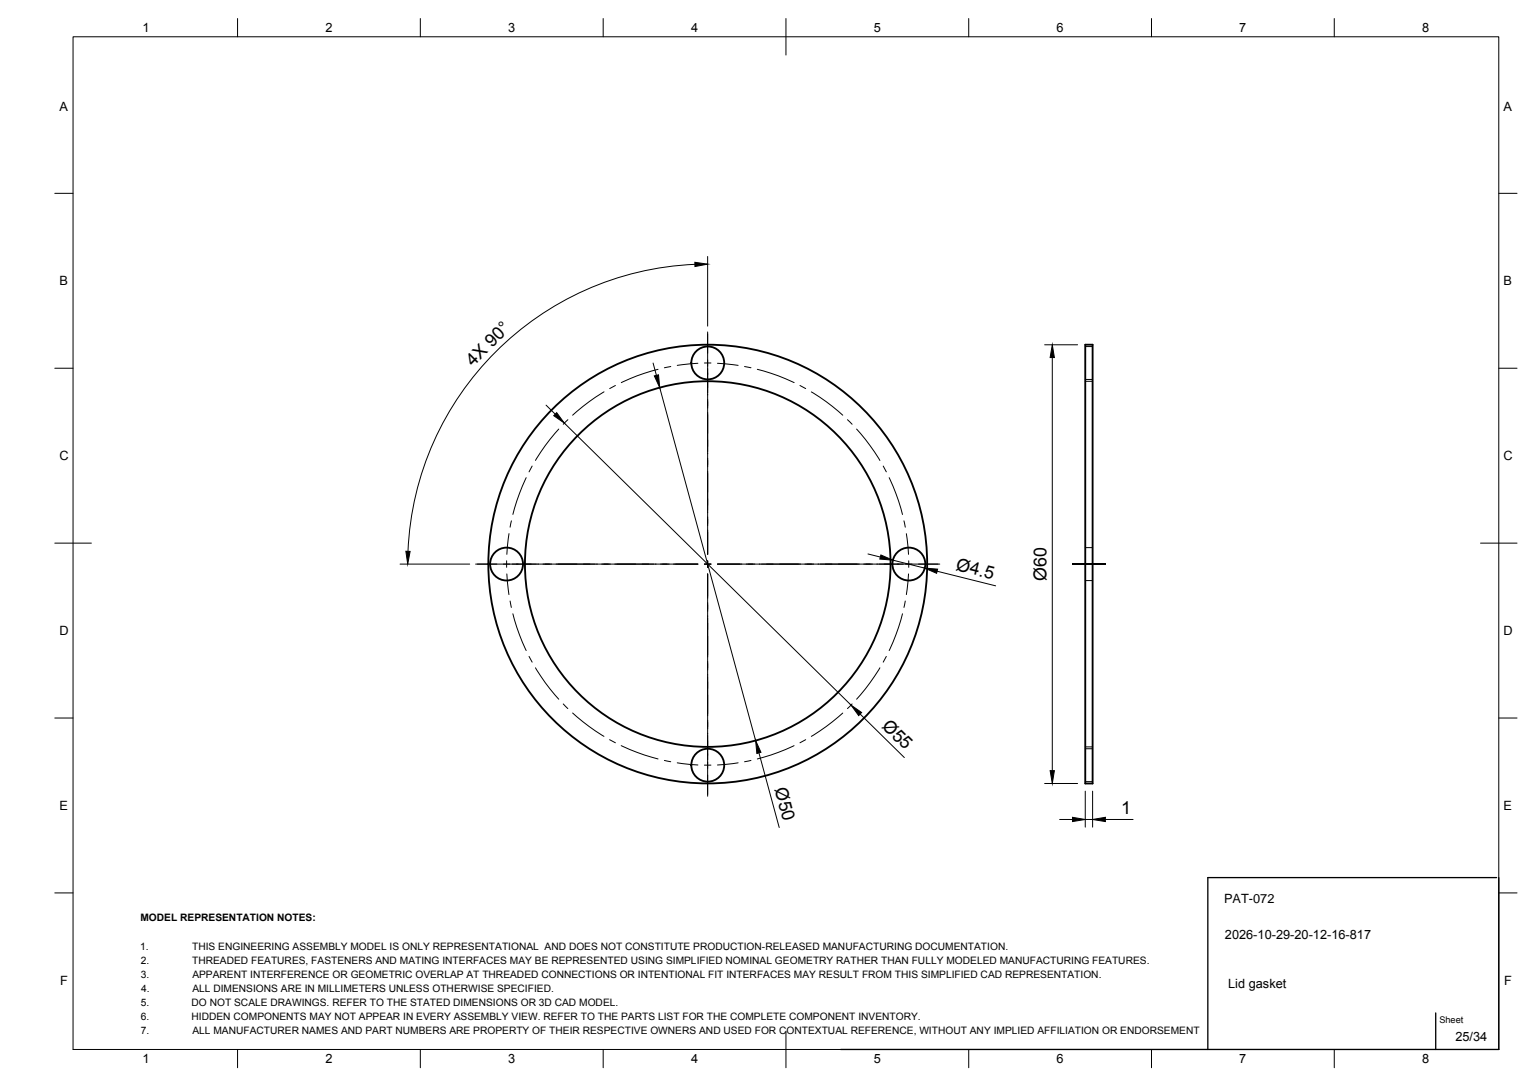
ISO-10303-21;
HEADER;
/* Generated by software containing ST-Developer
 * from STEP Tools, Inc. (www.steptools.com) 
 */

FILE_DESCRIPTION(
/* description */ ('PAT-072'),
/* implementation_level */ '2;1');

FILE_NAME(
/* name */ 'Lid gasket.step',
/* time_stamp */ '2026-10-29T20:11:56-07:00',
/* author */ (''),
/* organization */ (''),
/* preprocessor_version */ 'ST-DEVELOPER v20.2',
/* originating_system */ 'Autodesk Translation Framework v15.17.0.0',
/* authorisation */ '');

FILE_SCHEMA (('AUTOMOTIVE_DESIGN { 1 0 10303 214 3 1 1 }'));
ENDSEC;

DATA;
#10=MECHANICAL_DESIGN_GEOMETRIC_PRESENTATION_REPRESENTATION('',(#358),#11432);
#286=SHAPE_REPRESENTATION_RELATIONSHIP('SRR','None',#11590,#322);
#322=ADVANCED_BREP_SHAPE_REPRESENTATION('',(#394),#11421);
#358=STYLED_ITEM('',(#11833),#394);
#394=MANIFOLD_SOLID_BREP('Body1',#6093);
#532=FACE_BOUND('',#1572,.T.);
#533=FACE_BOUND('',#1573,.T.);
#534=FACE_BOUND('',#1574,.T.);
#535=FACE_BOUND('',#1575,.T.);
#536=FACE_BOUND('',#1576,.T.);
#537=FACE_BOUND('',#1578,.T.);
#538=FACE_BOUND('',#1579,.T.);
#539=FACE_BOUND('',#1580,.T.);
#540=FACE_BOUND('',#1581,.T.);
#541=FACE_BOUND('',#1582,.T.);
#730=PLANE('',#7043);
#731=PLANE('',#7044);
#1063=FACE_OUTER_BOUND('',#1565,.T.);
#1064=FACE_OUTER_BOUND('',#1566,.T.);
#1065=FACE_OUTER_BOUND('',#1567,.T.);
#1066=FACE_OUTER_BOUND('',#1568,.T.);
#1067=FACE_OUTER_BOUND('',#1569,.T.);
#1068=FACE_OUTER_BOUND('',#1570,.T.);
#1069=FACE_OUTER_BOUND('',#1571,.T.);
#1070=FACE_OUTER_BOUND('',#1577,.T.);
#1565=EDGE_LOOP('',(#5150,#5151,#5152,#5153));
#1566=EDGE_LOOP('',(#5154,#5155,#5156,#5157));
#1567=EDGE_LOOP('',(#5158,#5159,#5160,#5161));
#1568=EDGE_LOOP('',(#5162,#5163,#5164,#5165));
#1569=EDGE_LOOP('',(#5166,#5167,#5168,#5169));
#1570=EDGE_LOOP('',(#5170,#5171,#5172,#5173));
#1571=EDGE_LOOP('',(#5174));
#1572=EDGE_LOOP('',(#5175));
#1573=EDGE_LOOP('',(#5176));
#1574=EDGE_LOOP('',(#5177));
#1575=EDGE_LOOP('',(#5178));
#1576=EDGE_LOOP('',(#5179));
#1577=EDGE_LOOP('',(#5180));
#1578=EDGE_LOOP('',(#5181));
#1579=EDGE_LOOP('',(#5182));
#1580=EDGE_LOOP('',(#5183));
#1581=EDGE_LOOP('',(#5184));
#1582=EDGE_LOOP('',(#5185));
#1992=LINE('',#10857,#2411);
#1993=LINE('',#10863,#2412);
#1994=LINE('',#10869,#2413);
#1995=LINE('',#10875,#2414);
#1996=LINE('',#10881,#2415);
#1997=LINE('',#10887,#2416);
#2411=VECTOR('',#8593,0.225);
#2412=VECTOR('',#8600,0.225);
#2413=VECTOR('',#8607,0.225);
#2414=VECTOR('',#8614,0.225);
#2415=VECTOR('',#8621,2.5);
#2416=VECTOR('',#8628,3.);
#2767=CIRCLE('',#7026,0.225);
#2768=CIRCLE('',#7027,0.225);
#2769=CIRCLE('',#7029,0.225);
#2770=CIRCLE('',#7030,0.225);
#2771=CIRCLE('',#7032,0.225);
#2772=CIRCLE('',#7033,0.225);
#2773=CIRCLE('',#7035,0.225);
#2774=CIRCLE('',#7036,0.225);
#2775=CIRCLE('',#7038,2.5);
#2776=CIRCLE('',#7039,2.5);
#2777=CIRCLE('',#7041,3.);
#2778=CIRCLE('',#7042,3.);
#3190=VERTEX_POINT('',#10854);
#3191=VERTEX_POINT('',#10856);
#3192=VERTEX_POINT('',#10860);
#3193=VERTEX_POINT('',#10862);
#3194=VERTEX_POINT('',#10866);
#3195=VERTEX_POINT('',#10868);
#3196=VERTEX_POINT('',#10872);
#3197=VERTEX_POINT('',#10874);
#3198=VERTEX_POINT('',#10878);
#3199=VERTEX_POINT('',#10880);
#3200=VERTEX_POINT('',#10884);
#3201=VERTEX_POINT('',#10886);
#3864=EDGE_CURVE('',#3190,#3190,#2767,.T.);
#3865=EDGE_CURVE('',#3190,#3191,#1992,.T.);
#3866=EDGE_CURVE('',#3191,#3191,#2768,.T.);
#3867=EDGE_CURVE('',#3192,#3192,#2769,.T.);
#3868=EDGE_CURVE('',#3192,#3193,#1993,.T.);
#3869=EDGE_CURVE('',#3193,#3193,#2770,.T.);
#3870=EDGE_CURVE('',#3194,#3194,#2771,.T.);
#3871=EDGE_CURVE('',#3194,#3195,#1994,.T.);
#3872=EDGE_CURVE('',#3195,#3195,#2772,.T.);
#3873=EDGE_CURVE('',#3196,#3196,#2773,.T.);
#3874=EDGE_CURVE('',#3196,#3197,#1995,.T.);
#3875=EDGE_CURVE('',#3197,#3197,#2774,.T.);
#3876=EDGE_CURVE('',#3198,#3198,#2775,.T.);
#3877=EDGE_CURVE('',#3198,#3199,#1996,.T.);
#3878=EDGE_CURVE('',#3199,#3199,#2776,.T.);
#3879=EDGE_CURVE('',#3200,#3200,#2777,.T.);
#3880=EDGE_CURVE('',#3200,#3201,#1997,.T.);
#3881=EDGE_CURVE('',#3201,#3201,#2778,.T.);
#5150=ORIENTED_EDGE('',*,*,#3864,.F.);
#5151=ORIENTED_EDGE('',*,*,#3865,.T.);
#5152=ORIENTED_EDGE('',*,*,#3866,.F.);
#5153=ORIENTED_EDGE('',*,*,#3865,.F.);
#5154=ORIENTED_EDGE('',*,*,#3867,.F.);
#5155=ORIENTED_EDGE('',*,*,#3868,.T.);
#5156=ORIENTED_EDGE('',*,*,#3869,.F.);
#5157=ORIENTED_EDGE('',*,*,#3868,.F.);
#5158=ORIENTED_EDGE('',*,*,#3870,.F.);
#5159=ORIENTED_EDGE('',*,*,#3871,.T.);
#5160=ORIENTED_EDGE('',*,*,#3872,.F.);
#5161=ORIENTED_EDGE('',*,*,#3871,.F.);
#5162=ORIENTED_EDGE('',*,*,#3873,.F.);
#5163=ORIENTED_EDGE('',*,*,#3874,.T.);
#5164=ORIENTED_EDGE('',*,*,#3875,.F.);
#5165=ORIENTED_EDGE('',*,*,#3874,.F.);
#5166=ORIENTED_EDGE('',*,*,#3876,.F.);
#5167=ORIENTED_EDGE('',*,*,#3877,.T.);
#5168=ORIENTED_EDGE('',*,*,#3878,.T.);
#5169=ORIENTED_EDGE('',*,*,#3877,.F.);
#5170=ORIENTED_EDGE('',*,*,#3879,.F.);
#5171=ORIENTED_EDGE('',*,*,#3880,.T.);
#5172=ORIENTED_EDGE('',*,*,#3881,.T.);
#5173=ORIENTED_EDGE('',*,*,#3880,.F.);
#5174=ORIENTED_EDGE('',*,*,#3879,.T.);
#5175=ORIENTED_EDGE('',*,*,#3876,.T.);
#5176=ORIENTED_EDGE('',*,*,#3875,.T.);
#5177=ORIENTED_EDGE('',*,*,#3872,.T.);
#5178=ORIENTED_EDGE('',*,*,#3869,.T.);
#5179=ORIENTED_EDGE('',*,*,#3866,.T.);
#5180=ORIENTED_EDGE('',*,*,#3881,.F.);
#5181=ORIENTED_EDGE('',*,*,#3878,.F.);
#5182=ORIENTED_EDGE('',*,*,#3873,.T.);
#5183=ORIENTED_EDGE('',*,*,#3870,.T.);
#5184=ORIENTED_EDGE('',*,*,#3867,.T.);
#5185=ORIENTED_EDGE('',*,*,#3864,.T.);
#5665=CYLINDRICAL_SURFACE('',#7025,0.225);
#5666=CYLINDRICAL_SURFACE('',#7028,0.225);
#5667=CYLINDRICAL_SURFACE('',#7031,0.225);
#5668=CYLINDRICAL_SURFACE('',#7034,0.225);
#5669=CYLINDRICAL_SURFACE('',#7037,2.5);
#5670=CYLINDRICAL_SURFACE('',#7040,3.);
#5962=ADVANCED_FACE('',(#1063),#5665,.F.);
#5963=ADVANCED_FACE('',(#1064),#5666,.F.);
#5964=ADVANCED_FACE('',(#1065),#5667,.F.);
#5965=ADVANCED_FACE('',(#1066),#5668,.F.);
#5966=ADVANCED_FACE('',(#1067),#5669,.F.);
#5967=ADVANCED_FACE('',(#1068),#5670,.T.);
#5968=ADVANCED_FACE('',(#1069,#532,#533,#534,#535,#536),#730,.T.);
#5969=ADVANCED_FACE('',(#1070,#537,#538,#539,#540,#541),#731,.F.);
#6093=CLOSED_SHELL('',(#5962,#5963,#5964,#5965,#5966,#5967,#5968,#5969));
#7024=AXIS2_PLACEMENT_3D('',#10852,#8587,#8588);
#7025=AXIS2_PLACEMENT_3D('',#10853,#8589,#8590);
#7026=AXIS2_PLACEMENT_3D('',#10855,#8591,#8592);
#7027=AXIS2_PLACEMENT_3D('',#10858,#8594,#8595);
#7028=AXIS2_PLACEMENT_3D('',#10859,#8596,#8597);
#7029=AXIS2_PLACEMENT_3D('',#10861,#8598,#8599);
#7030=AXIS2_PLACEMENT_3D('',#10864,#8601,#8602);
#7031=AXIS2_PLACEMENT_3D('',#10865,#8603,#8604);
#7032=AXIS2_PLACEMENT_3D('',#10867,#8605,#8606);
#7033=AXIS2_PLACEMENT_3D('',#10870,#8608,#8609);
#7034=AXIS2_PLACEMENT_3D('',#10871,#8610,#8611);
#7035=AXIS2_PLACEMENT_3D('',#10873,#8612,#8613);
#7036=AXIS2_PLACEMENT_3D('',#10876,#8615,#8616);
#7037=AXIS2_PLACEMENT_3D('',#10877,#8617,#8618);
#7038=AXIS2_PLACEMENT_3D('',#10879,#8619,#8620);
#7039=AXIS2_PLACEMENT_3D('',#10882,#8622,#8623);
#7040=AXIS2_PLACEMENT_3D('',#10883,#8624,#8625);
#7041=AXIS2_PLACEMENT_3D('',#10885,#8626,#8627);
#7042=AXIS2_PLACEMENT_3D('',#10888,#8629,#8630);
#7043=AXIS2_PLACEMENT_3D('',#10889,#8631,#8632);
#7044=AXIS2_PLACEMENT_3D('',#10890,#8633,#8634);
#8587=DIRECTION('axis',(0.,0.,1.));
#8588=DIRECTION('refdir',(1.,0.,0.));
#8589=DIRECTION('center_axis',(0.,0.,1.));
#8590=DIRECTION('ref_axis',(1.,0.,0.));
#8591=DIRECTION('center_axis',(0.,0.,1.));
#8592=DIRECTION('ref_axis',(1.,0.,0.));
#8593=DIRECTION('',(0.,0.,1.));
#8594=DIRECTION('center_axis',(0.,0.,-1.));
#8595=DIRECTION('ref_axis',(1.,0.,0.));
#8596=DIRECTION('center_axis',(0.,0.,1.));
#8597=DIRECTION('ref_axis',(1.,0.,0.));
#8598=DIRECTION('center_axis',(0.,0.,1.));
#8599=DIRECTION('ref_axis',(1.,0.,0.));
#8600=DIRECTION('',(0.,0.,1.));
#8601=DIRECTION('center_axis',(0.,0.,-1.));
#8602=DIRECTION('ref_axis',(1.,0.,0.));
#8603=DIRECTION('center_axis',(0.,0.,1.));
#8604=DIRECTION('ref_axis',(1.,0.,0.));
#8605=DIRECTION('center_axis',(0.,0.,1.));
#8606=DIRECTION('ref_axis',(1.,0.,0.));
#8607=DIRECTION('',(0.,0.,1.));
#8608=DIRECTION('center_axis',(0.,0.,-1.));
#8609=DIRECTION('ref_axis',(1.,0.,0.));
#8610=DIRECTION('center_axis',(0.,0.,1.));
#8611=DIRECTION('ref_axis',(1.,0.,0.));
#8612=DIRECTION('center_axis',(0.,0.,1.));
#8613=DIRECTION('ref_axis',(1.,0.,0.));
#8614=DIRECTION('',(0.,0.,1.));
#8615=DIRECTION('center_axis',(0.,0.,-1.));
#8616=DIRECTION('ref_axis',(1.,0.,0.));
#8617=DIRECTION('center_axis',(0.,0.,1.));
#8618=DIRECTION('ref_axis',(1.,0.,0.));
#8619=DIRECTION('center_axis',(0.,0.,-1.));
#8620=DIRECTION('ref_axis',(1.,0.,0.));
#8621=DIRECTION('',(0.,0.,-1.));
#8622=DIRECTION('center_axis',(0.,0.,-1.));
#8623=DIRECTION('ref_axis',(1.,0.,0.));
#8624=DIRECTION('center_axis',(0.,0.,1.));
#8625=DIRECTION('ref_axis',(1.,0.,0.));
#8626=DIRECTION('center_axis',(0.,0.,1.));
#8627=DIRECTION('ref_axis',(1.,0.,0.));
#8628=DIRECTION('',(0.,0.,-1.));
#8629=DIRECTION('center_axis',(0.,0.,1.));
#8630=DIRECTION('ref_axis',(1.,0.,0.));
#8631=DIRECTION('center_axis',(0.,0.,1.));
#8632=DIRECTION('ref_axis',(1.,0.,0.));
#8633=DIRECTION('center_axis',(0.,0.,1.));
#8634=DIRECTION('ref_axis',(1.,0.,0.));
#10852=CARTESIAN_POINT('',(0.,0.,0.));
#10853=CARTESIAN_POINT('Origin',(-2.75,3.36777869765522E-16,14.9));
#10854=CARTESIAN_POINT('',(-2.975,3.09223316784707E-16,15.));
#10855=CARTESIAN_POINT('Origin',(-2.75,3.36777869765522E-16,15.));
#10856=CARTESIAN_POINT('',(-2.975,3.64332422746338E-16,15.1));
#10857=CARTESIAN_POINT('',(-2.975,3.09223316784707E-16,14.9));
#10858=CARTESIAN_POINT('Origin',(-2.75,3.36777869765522E-16,15.1));
#10859=CARTESIAN_POINT('Origin',(1.68388934882761E-16,2.75,14.9));
#10860=CARTESIAN_POINT('',(-0.225,2.75,15.));
#10861=CARTESIAN_POINT('Origin',(1.68388934882761E-16,2.75,15.));
#10862=CARTESIAN_POINT('',(-0.225,2.75,15.1));
#10863=CARTESIAN_POINT('',(-0.225,2.75,14.9));
#10864=CARTESIAN_POINT('Origin',(1.68388934882761E-16,2.75,15.1));
#10865=CARTESIAN_POINT('Origin',(2.75,0.,14.9));
#10866=CARTESIAN_POINT('',(2.525,-2.75545529808155E-17,15.));
#10867=CARTESIAN_POINT('Origin',(2.75,0.,15.));
#10868=CARTESIAN_POINT('',(2.525,2.75545529808155E-17,15.1));
#10869=CARTESIAN_POINT('',(2.525,-2.75545529808155E-17,14.9));
#10870=CARTESIAN_POINT('Origin',(2.75,0.,15.1));
#10871=CARTESIAN_POINT('Origin',(-5.05166804648283E-16,-2.75,14.9));
#10872=CARTESIAN_POINT('',(-0.225000000000001,-2.75,15.));
#10873=CARTESIAN_POINT('Origin',(-5.05166804648283E-16,-2.75,15.));
#10874=CARTESIAN_POINT('',(-0.225000000000001,-2.75,15.1));
#10875=CARTESIAN_POINT('',(-0.225000000000001,-2.75,14.9));
#10876=CARTESIAN_POINT('Origin',(-5.05166804648283E-16,-2.75,15.1));
#10877=CARTESIAN_POINT('Origin',(0.,0.,15.));
#10878=CARTESIAN_POINT('',(-2.5,-3.06161699786838E-16,15.1));
#10879=CARTESIAN_POINT('Origin',(0.,0.,15.1));
#10880=CARTESIAN_POINT('',(-2.5,-3.06161699786838E-16,15.));
#10881=CARTESIAN_POINT('',(-2.5,-3.06161699786838E-16,15.));
#10882=CARTESIAN_POINT('Origin',(0.,0.,15.));
#10883=CARTESIAN_POINT('Origin',(0.,0.,15.));
#10884=CARTESIAN_POINT('',(-3.,-3.67394039744206E-16,15.1));
#10885=CARTESIAN_POINT('Origin',(0.,0.,15.1));
#10886=CARTESIAN_POINT('',(-3.,-3.67394039744206E-16,15.));
#10887=CARTESIAN_POINT('',(-3.,-3.67394039744206E-16,15.));
#10888=CARTESIAN_POINT('Origin',(0.,0.,15.));
#10889=CARTESIAN_POINT('Origin',(0.,0.,15.1));
#10890=CARTESIAN_POINT('Origin',(0.,0.,15.));
#11382=UNCERTAINTY_MEASURE_WITH_UNIT(LENGTH_MEASURE(0.001),#11433,
'DISTANCE_ACCURACY_VALUE',
'Maximum model space distance between geometric entities at asserted c
onnectivities');
#11393=UNCERTAINTY_MEASURE_WITH_UNIT(LENGTH_MEASURE(0.001),#11433,
'DISTANCE_ACCURACY_VALUE',
'Maximum model space distance between geometric entities at asserted c
onnectivities');
#11421=(
GEOMETRIC_REPRESENTATION_CONTEXT(3)
GLOBAL_UNCERTAINTY_ASSIGNED_CONTEXT((#11382))
GLOBAL_UNIT_ASSIGNED_CONTEXT((#11433,#11435,#11436))
REPRESENTATION_CONTEXT('','3D')
);
#11432=(
GEOMETRIC_REPRESENTATION_CONTEXT(3)
GLOBAL_UNCERTAINTY_ASSIGNED_CONTEXT((#11393))
GLOBAL_UNIT_ASSIGNED_CONTEXT((#11433,#11435,#11436))
REPRESENTATION_CONTEXT('','3D')
);
#11433=(
LENGTH_UNIT()
NAMED_UNIT(*)
SI_UNIT(.CENTI.,.METRE.)
);
#11435=(
NAMED_UNIT(*)
PLANE_ANGLE_UNIT()
SI_UNIT($,.RADIAN.)
);
#11436=(
NAMED_UNIT(*)
SI_UNIT($,.STERADIAN.)
SOLID_ANGLE_UNIT()
);
#11464=SHAPE_DEFINITION_REPRESENTATION(#11502,#11590);
#11502=PRODUCT_DEFINITION_SHAPE('',$,#11629);
#11590=SHAPE_REPRESENTATION('',(#7024),#11421);
#11601=PRODUCT_DEFINITION_CONTEXT('part definition',#11717,'design');
#11629=PRODUCT_DEFINITION('Lid gasket','Lid gasket',#11667,
#11601);
#11667=PRODUCT_DEFINITION_FORMATION('',$,#11746);
#11717=APPLICATION_CONTEXT(
'Core Data for Automotive Mechanical Design Process');
#11718=PRODUCT_CONTEXT('part definition',#11717,'mechanical');
#11746=PRODUCT('Lid gasket','Lid gasket','Lid gasket',(#11718));
#11827=COLOUR_RGB('Off White',0.89,0.88,0.83);
#11828=FILL_AREA_STYLE_COLOUR('',#11827);
#11829=FILL_AREA_STYLE('',(#11828));
#11830=SURFACE_STYLE_FILL_AREA(#11829);
#11831=SURFACE_SIDE_STYLE('',(#11830));
#11832=SURFACE_STYLE_USAGE(.BOTH.,#11831);
#11833=PRESENTATION_STYLE_ASSIGNMENT((#11832));
ENDSEC;
END-ISO-10303-21;
